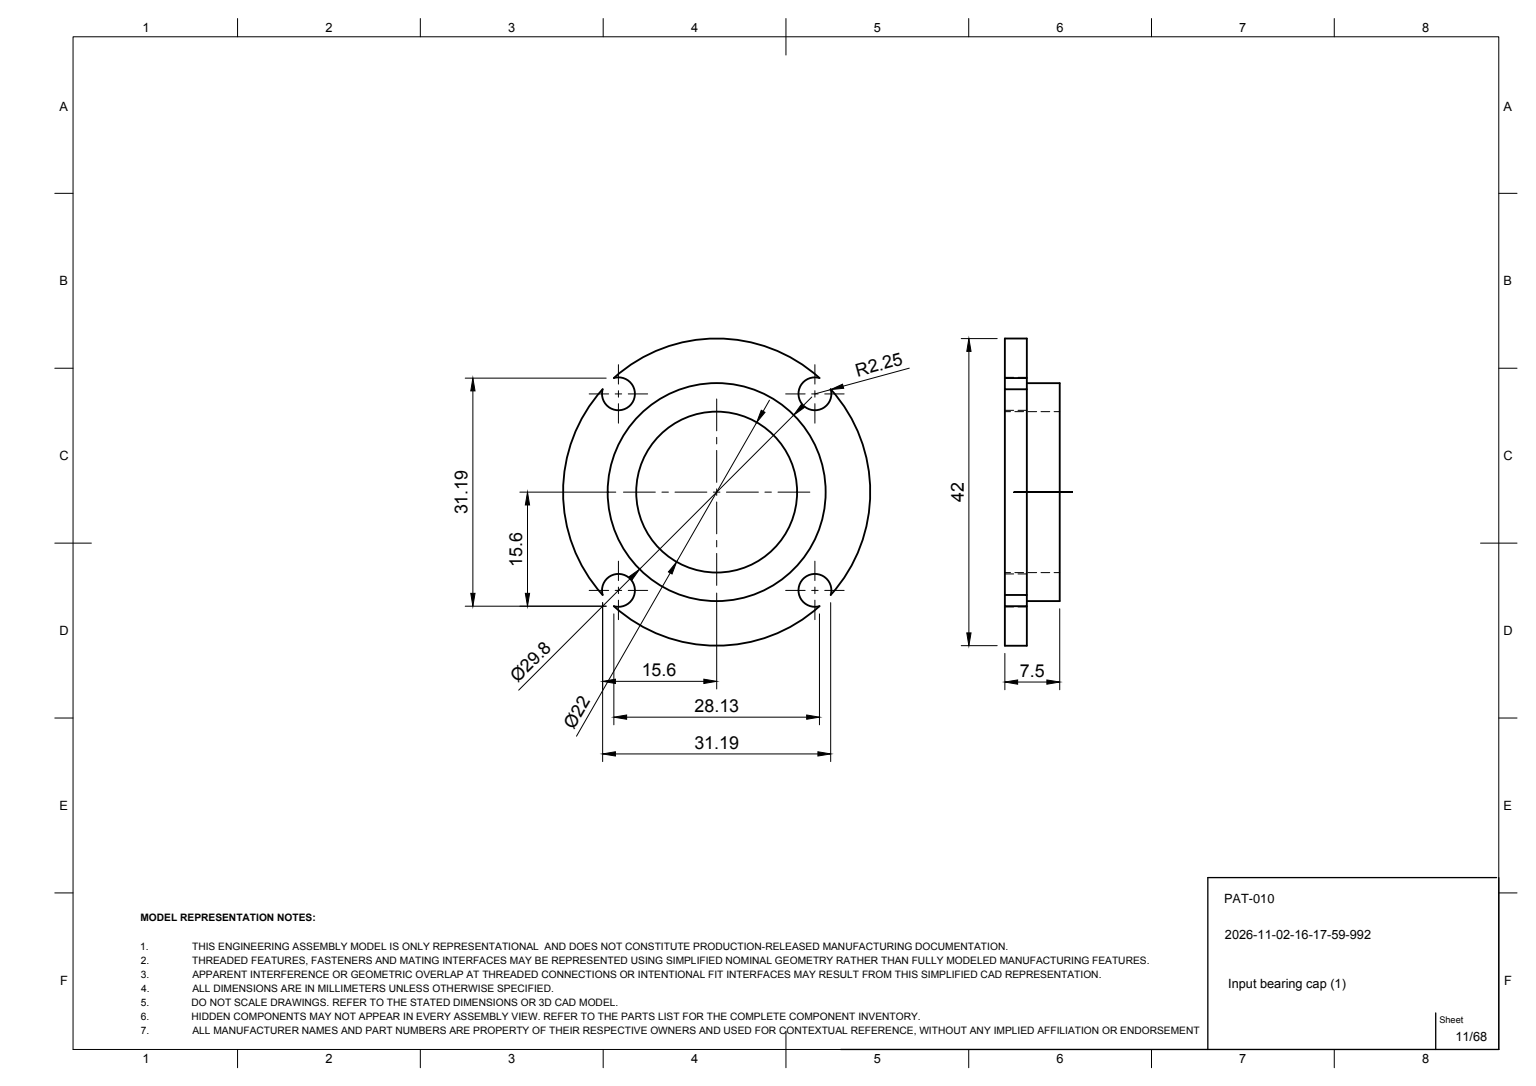
ISO-10303-21;
HEADER;
/* Generated by software containing ST-Developer
 * from STEP Tools, Inc. (www.steptools.com) 
 */

FILE_DESCRIPTION(
/* description */ ('Belt conveyor head drive unit'),
/* implementation_level */ '2;1');

FILE_NAME(
/* name */ 'Input bearing cap (1).step',
/* time_stamp */ '2026-10-28T03:26:19-07:00',
/* author */ (''),
/* organization */ (''),
/* preprocessor_version */ 'ST-DEVELOPER v20.2',
/* originating_system */ 'Autodesk Translation Framework v15.17.0.0',
/* authorisation */ '');

FILE_SCHEMA (('AUTOMOTIVE_DESIGN { 1 0 10303 214 3 1 1 }'));
ENDSEC;

DATA;
#10=MECHANICAL_DESIGN_GEOMETRIC_PRESENTATION_REPRESENTATION('',(#853),#27069);
#715=SHAPE_REPRESENTATION_RELATIONSHIP('SRR','None',#27359,#784);
#784=ADVANCED_BREP_SHAPE_REPRESENTATION('',(#938),#27001);
#853=STYLED_ITEM('',(#27797),#938);
#938=MANIFOLD_SOLID_BREP('Body1',#13718);
#1055=FACE_BOUND('',#2579,.T.);
#1056=FACE_BOUND('',#2586,.T.);
#1057=FACE_BOUND('',#2589,.T.);
#1332=PLANE('',#14771);
#1333=PLANE('',#14787);
#1334=PLANE('',#14791);
#1731=FACE_OUTER_BOUND('',#2574,.T.);
#1732=FACE_OUTER_BOUND('',#2575,.T.);
#1733=FACE_OUTER_BOUND('',#2576,.T.);
#1734=FACE_OUTER_BOUND('',#2577,.T.);
#1735=FACE_OUTER_BOUND('',#2578,.T.);
#1736=FACE_OUTER_BOUND('',#2580,.T.);
#1737=FACE_OUTER_BOUND('',#2581,.T.);
#1738=FACE_OUTER_BOUND('',#2582,.T.);
#1739=FACE_OUTER_BOUND('',#2583,.T.);
#1740=FACE_OUTER_BOUND('',#2584,.T.);
#1741=FACE_OUTER_BOUND('',#2585,.T.);
#1742=FACE_OUTER_BOUND('',#2587,.T.);
#1743=FACE_OUTER_BOUND('',#2588,.T.);
#2574=EDGE_LOOP('',(#9396,#9397,#9398,#9399));
#2575=EDGE_LOOP('',(#9400,#9401,#9402,#9403));
#2576=EDGE_LOOP('',(#9404,#9405,#9406,#9407));
#2577=EDGE_LOOP('',(#9408,#9409,#9410,#9411));
#2578=EDGE_LOOP('',(#9412,#9413,#9414,#9415,#9416,#9417,#9418,#9419));
#2579=EDGE_LOOP('',(#9420));
#2580=EDGE_LOOP('',(#9421,#9422,#9423,#9424));
#2581=EDGE_LOOP('',(#9425,#9426,#9427,#9428));
#2582=EDGE_LOOP('',(#9429,#9430,#9431,#9432));
#2583=EDGE_LOOP('',(#9433,#9434,#9435,#9436));
#2584=EDGE_LOOP('',(#9437,#9438,#9439,#9440));
#2585=EDGE_LOOP('',(#9441));
#2586=EDGE_LOOP('',(#9442));
#2587=EDGE_LOOP('',(#9443,#9444,#9445,#9446));
#2588=EDGE_LOOP('',(#9447,#9448,#9449,#9450,#9451,#9452,#9453,#9454));
#2589=EDGE_LOOP('',(#9455));
#3627=LINE('',#21445,#4419);
#3628=LINE('',#21449,#4420);
#3629=LINE('',#21454,#4421);
#3630=LINE('',#21458,#4422);
#3631=LINE('',#21463,#4423);
#3632=LINE('',#21467,#4424);
#3633=LINE('',#21472,#4425);
#3634=LINE('',#21476,#4426);
#3635=LINE('',#21495,#4427);
#3636=LINE('',#21503,#4428);
#4419=VECTOR('',#16959,1.);
#4420=VECTOR('',#16962,1.);
#4421=VECTOR('',#16967,1.);
#4422=VECTOR('',#16970,1.);
#4423=VECTOR('',#16975,1.);
#4424=VECTOR('',#16978,1.);
#4425=VECTOR('',#16983,1.);
#4426=VECTOR('',#16986,1.);
#4427=VECTOR('',#17019,1.49);
#4428=VECTOR('',#17030,1.1);
#5172=CIRCLE('',#14760,0.225);
#5173=CIRCLE('',#14761,0.225);
#5174=CIRCLE('',#14763,0.225);
#5175=CIRCLE('',#14764,0.225);
#5176=CIRCLE('',#14766,0.225);
#5177=CIRCLE('',#14767,0.225);
#5178=CIRCLE('',#14769,0.225);
#5179=CIRCLE('',#14770,0.225);
#5180=CIRCLE('',#14772,2.1);
#5181=CIRCLE('',#14773,2.1);
#5182=CIRCLE('',#14774,2.1);
#5183=CIRCLE('',#14775,2.1);
#5184=CIRCLE('',#14776,1.49);
#5185=CIRCLE('',#14778,2.1);
#5186=CIRCLE('',#14780,2.1);
#5187=CIRCLE('',#14782,2.1);
#5188=CIRCLE('',#14784,2.1);
#5189=CIRCLE('',#14786,1.49);
#5190=CIRCLE('',#14788,1.1);
#5191=CIRCLE('',#14790,1.1);
#6099=VERTEX_POINT('',#21443);
#6100=VERTEX_POINT('',#21444);
#6101=VERTEX_POINT('',#21446);
#6102=VERTEX_POINT('',#21448);
#6103=VERTEX_POINT('',#21452);
#6104=VERTEX_POINT('',#21453);
#6105=VERTEX_POINT('',#21455);
#6106=VERTEX_POINT('',#21457);
#6107=VERTEX_POINT('',#21461);
#6108=VERTEX_POINT('',#21462);
#6109=VERTEX_POINT('',#21464);
#6110=VERTEX_POINT('',#21466);
#6111=VERTEX_POINT('',#21470);
#6112=VERTEX_POINT('',#21471);
#6113=VERTEX_POINT('',#21473);
#6114=VERTEX_POINT('',#21475);
#6115=VERTEX_POINT('',#21483);
#6116=VERTEX_POINT('',#21494);
#6117=VERTEX_POINT('',#21498);
#6118=VERTEX_POINT('',#21501);
#7390=EDGE_CURVE('',#6099,#6100,#3627,.T.);
#7391=EDGE_CURVE('',#6101,#6099,#5172,.T.);
#7392=EDGE_CURVE('',#6102,#6101,#3628,.T.);
#7393=EDGE_CURVE('',#6100,#6102,#5173,.T.);
#7394=EDGE_CURVE('',#6103,#6104,#3629,.T.);
#7395=EDGE_CURVE('',#6105,#6103,#5174,.T.);
#7396=EDGE_CURVE('',#6106,#6105,#3630,.T.);
#7397=EDGE_CURVE('',#6104,#6106,#5175,.T.);
#7398=EDGE_CURVE('',#6107,#6108,#3631,.T.);
#7399=EDGE_CURVE('',#6109,#6107,#5176,.T.);
#7400=EDGE_CURVE('',#6110,#6109,#3632,.T.);
#7401=EDGE_CURVE('',#6108,#6110,#5177,.T.);
#7402=EDGE_CURVE('',#6111,#6112,#3633,.T.);
#7403=EDGE_CURVE('',#6113,#6111,#5178,.T.);
#7404=EDGE_CURVE('',#6114,#6113,#3634,.T.);
#7405=EDGE_CURVE('',#6112,#6114,#5179,.T.);
#7406=EDGE_CURVE('',#6113,#6099,#5180,.T.);
#7407=EDGE_CURVE('',#6109,#6111,#5181,.T.);
#7408=EDGE_CURVE('',#6105,#6107,#5182,.T.);
#7409=EDGE_CURVE('',#6101,#6103,#5183,.T.);
#7410=EDGE_CURVE('',#6115,#6115,#5184,.T.);
#7411=EDGE_CURVE('',#6110,#6112,#5185,.T.);
#7412=EDGE_CURVE('',#6106,#6108,#5186,.T.);
#7413=EDGE_CURVE('',#6114,#6100,#5187,.T.);
#7414=EDGE_CURVE('',#6102,#6104,#5188,.T.);
#7415=EDGE_CURVE('',#6115,#6116,#3635,.T.);
#7416=EDGE_CURVE('',#6116,#6116,#5189,.T.);
#7417=EDGE_CURVE('',#6117,#6117,#5190,.T.);
#7418=EDGE_CURVE('',#6118,#6118,#5191,.T.);
#7419=EDGE_CURVE('',#6118,#6117,#3636,.T.);
#9396=ORIENTED_EDGE('',*,*,#7390,.F.);
#9397=ORIENTED_EDGE('',*,*,#7391,.F.);
#9398=ORIENTED_EDGE('',*,*,#7392,.F.);
#9399=ORIENTED_EDGE('',*,*,#7393,.F.);
#9400=ORIENTED_EDGE('',*,*,#7394,.F.);
#9401=ORIENTED_EDGE('',*,*,#7395,.F.);
#9402=ORIENTED_EDGE('',*,*,#7396,.F.);
#9403=ORIENTED_EDGE('',*,*,#7397,.F.);
#9404=ORIENTED_EDGE('',*,*,#7398,.F.);
#9405=ORIENTED_EDGE('',*,*,#7399,.F.);
#9406=ORIENTED_EDGE('',*,*,#7400,.F.);
#9407=ORIENTED_EDGE('',*,*,#7401,.F.);
#9408=ORIENTED_EDGE('',*,*,#7402,.F.);
#9409=ORIENTED_EDGE('',*,*,#7403,.F.);
#9410=ORIENTED_EDGE('',*,*,#7404,.F.);
#9411=ORIENTED_EDGE('',*,*,#7405,.F.);
#9412=ORIENTED_EDGE('',*,*,#7391,.T.);
#9413=ORIENTED_EDGE('',*,*,#7406,.F.);
#9414=ORIENTED_EDGE('',*,*,#7403,.T.);
#9415=ORIENTED_EDGE('',*,*,#7407,.F.);
#9416=ORIENTED_EDGE('',*,*,#7399,.T.);
#9417=ORIENTED_EDGE('',*,*,#7408,.F.);
#9418=ORIENTED_EDGE('',*,*,#7395,.T.);
#9419=ORIENTED_EDGE('',*,*,#7409,.F.);
#9420=ORIENTED_EDGE('',*,*,#7410,.T.);
#9421=ORIENTED_EDGE('',*,*,#7400,.T.);
#9422=ORIENTED_EDGE('',*,*,#7407,.T.);
#9423=ORIENTED_EDGE('',*,*,#7402,.T.);
#9424=ORIENTED_EDGE('',*,*,#7411,.F.);
#9425=ORIENTED_EDGE('',*,*,#7396,.T.);
#9426=ORIENTED_EDGE('',*,*,#7408,.T.);
#9427=ORIENTED_EDGE('',*,*,#7398,.T.);
#9428=ORIENTED_EDGE('',*,*,#7412,.F.);
#9429=ORIENTED_EDGE('',*,*,#7390,.T.);
#9430=ORIENTED_EDGE('',*,*,#7413,.F.);
#9431=ORIENTED_EDGE('',*,*,#7404,.T.);
#9432=ORIENTED_EDGE('',*,*,#7406,.T.);
#9433=ORIENTED_EDGE('',*,*,#7392,.T.);
#9434=ORIENTED_EDGE('',*,*,#7409,.T.);
#9435=ORIENTED_EDGE('',*,*,#7394,.T.);
#9436=ORIENTED_EDGE('',*,*,#7414,.F.);
#9437=ORIENTED_EDGE('',*,*,#7410,.F.);
#9438=ORIENTED_EDGE('',*,*,#7415,.T.);
#9439=ORIENTED_EDGE('',*,*,#7416,.T.);
#9440=ORIENTED_EDGE('',*,*,#7415,.F.);
#9441=ORIENTED_EDGE('',*,*,#7416,.F.);
#9442=ORIENTED_EDGE('',*,*,#7417,.F.);
#9443=ORIENTED_EDGE('',*,*,#7418,.F.);
#9444=ORIENTED_EDGE('',*,*,#7419,.T.);
#9445=ORIENTED_EDGE('',*,*,#7417,.T.);
#9446=ORIENTED_EDGE('',*,*,#7419,.F.);
#9447=ORIENTED_EDGE('',*,*,#7393,.T.);
#9448=ORIENTED_EDGE('',*,*,#7414,.T.);
#9449=ORIENTED_EDGE('',*,*,#7397,.T.);
#9450=ORIENTED_EDGE('',*,*,#7412,.T.);
#9451=ORIENTED_EDGE('',*,*,#7401,.T.);
#9452=ORIENTED_EDGE('',*,*,#7411,.T.);
#9453=ORIENTED_EDGE('',*,*,#7405,.T.);
#9454=ORIENTED_EDGE('',*,*,#7413,.T.);
#9455=ORIENTED_EDGE('',*,*,#7418,.T.);
#12575=CYLINDRICAL_SURFACE('',#14759,0.225);
#12576=CYLINDRICAL_SURFACE('',#14762,0.225);
#12577=CYLINDRICAL_SURFACE('',#14765,0.225);
#12578=CYLINDRICAL_SURFACE('',#14768,0.225);
#12579=CYLINDRICAL_SURFACE('',#14777,2.1);
#12580=CYLINDRICAL_SURFACE('',#14779,2.1);
#12581=CYLINDRICAL_SURFACE('',#14781,2.1);
#12582=CYLINDRICAL_SURFACE('',#14783,2.1);
#12583=CYLINDRICAL_SURFACE('',#14785,1.49);
#12584=CYLINDRICAL_SURFACE('',#14789,1.1);
#13010=ADVANCED_FACE('',(#1731),#12575,.F.);
#13011=ADVANCED_FACE('',(#1732),#12576,.F.);
#13012=ADVANCED_FACE('',(#1733),#12577,.F.);
#13013=ADVANCED_FACE('',(#1734),#12578,.F.);
#13014=ADVANCED_FACE('',(#1735,#1055),#1332,.F.);
#13015=ADVANCED_FACE('',(#1736),#12579,.T.);
#13016=ADVANCED_FACE('',(#1737),#12580,.T.);
#13017=ADVANCED_FACE('',(#1738),#12581,.T.);
#13018=ADVANCED_FACE('',(#1739),#12582,.T.);
#13019=ADVANCED_FACE('',(#1740),#12583,.T.);
#13020=ADVANCED_FACE('',(#1741,#1056),#1333,.F.);
#13021=ADVANCED_FACE('',(#1742),#12584,.F.);
#13022=ADVANCED_FACE('',(#1743,#1057),#1334,.T.);
#13718=CLOSED_SHELL('',(#13010,#13011,#13012,#13013,#13014,#13015,#13016,
#13017,#13018,#13019,#13020,#13021,#13022));
#14758=AXIS2_PLACEMENT_3D('',#21441,#16955,#16956);
#14759=AXIS2_PLACEMENT_3D('',#21442,#16957,#16958);
#14760=AXIS2_PLACEMENT_3D('',#21447,#16960,#16961);
#14761=AXIS2_PLACEMENT_3D('',#21450,#16963,#16964);
#14762=AXIS2_PLACEMENT_3D('',#21451,#16965,#16966);
#14763=AXIS2_PLACEMENT_3D('',#21456,#16968,#16969);
#14764=AXIS2_PLACEMENT_3D('',#21459,#16971,#16972);
#14765=AXIS2_PLACEMENT_3D('',#21460,#16973,#16974);
#14766=AXIS2_PLACEMENT_3D('',#21465,#16976,#16977);
#14767=AXIS2_PLACEMENT_3D('',#21468,#16979,#16980);
#14768=AXIS2_PLACEMENT_3D('',#21469,#16981,#16982);
#14769=AXIS2_PLACEMENT_3D('',#21474,#16984,#16985);
#14770=AXIS2_PLACEMENT_3D('',#21477,#16987,#16988);
#14771=AXIS2_PLACEMENT_3D('',#21478,#16989,#16990);
#14772=AXIS2_PLACEMENT_3D('',#21479,#16991,#16992);
#14773=AXIS2_PLACEMENT_3D('',#21480,#16993,#16994);
#14774=AXIS2_PLACEMENT_3D('',#21481,#16995,#16996);
#14775=AXIS2_PLACEMENT_3D('',#21482,#16997,#16998);
#14776=AXIS2_PLACEMENT_3D('',#21484,#16999,#17000);
#14777=AXIS2_PLACEMENT_3D('',#21485,#17001,#17002);
#14778=AXIS2_PLACEMENT_3D('',#21486,#17003,#17004);
#14779=AXIS2_PLACEMENT_3D('',#21487,#17005,#17006);
#14780=AXIS2_PLACEMENT_3D('',#21488,#17007,#17008);
#14781=AXIS2_PLACEMENT_3D('',#21489,#17009,#17010);
#14782=AXIS2_PLACEMENT_3D('',#21490,#17011,#17012);
#14783=AXIS2_PLACEMENT_3D('',#21491,#17013,#17014);
#14784=AXIS2_PLACEMENT_3D('',#21492,#17015,#17016);
#14785=AXIS2_PLACEMENT_3D('',#21493,#17017,#17018);
#14786=AXIS2_PLACEMENT_3D('',#21496,#17020,#17021);
#14787=AXIS2_PLACEMENT_3D('',#21497,#17022,#17023);
#14788=AXIS2_PLACEMENT_3D('',#21499,#17024,#17025);
#14789=AXIS2_PLACEMENT_3D('',#21500,#17026,#17027);
#14790=AXIS2_PLACEMENT_3D('',#21502,#17028,#17029);
#14791=AXIS2_PLACEMENT_3D('',#21504,#17031,#17032);
#16955=DIRECTION('axis',(0.,0.,1.));
#16956=DIRECTION('refdir',(1.,0.,0.));
#16957=DIRECTION('center_axis',(0.,1.,0.));
#16958=DIRECTION('ref_axis',(0.707106781186546,0.,0.707106781186549));
#16959=DIRECTION('',(0.,1.,0.));
#16960=DIRECTION('center_axis',(0.,1.,0.));
#16961=DIRECTION('ref_axis',(1.,0.,0.));
#16962=DIRECTION('',(0.,-1.,0.));
#16963=DIRECTION('center_axis',(0.,-1.,0.));
#16964=DIRECTION('ref_axis',(1.,0.,0.));
#16965=DIRECTION('center_axis',(0.,1.,0.));
#16966=DIRECTION('ref_axis',(0.707106781186547,0.,-0.707106781186548));
#16967=DIRECTION('',(0.,1.,0.));
#16968=DIRECTION('center_axis',(0.,1.,0.));
#16969=DIRECTION('ref_axis',(1.,0.,0.));
#16970=DIRECTION('',(0.,-1.,0.));
#16971=DIRECTION('center_axis',(0.,-1.,0.));
#16972=DIRECTION('ref_axis',(1.,0.,0.));
#16973=DIRECTION('center_axis',(0.,1.,0.));
#16974=DIRECTION('ref_axis',(-0.707106781186552,0.,-0.707106781186543));
#16975=DIRECTION('',(0.,1.,0.));
#16976=DIRECTION('center_axis',(0.,1.,0.));
#16977=DIRECTION('ref_axis',(1.,0.,0.));
#16978=DIRECTION('',(0.,-1.,0.));
#16979=DIRECTION('center_axis',(0.,-1.,0.));
#16980=DIRECTION('ref_axis',(1.,0.,0.));
#16981=DIRECTION('center_axis',(0.,1.,0.));
#16982=DIRECTION('ref_axis',(-0.707106781186546,0.,0.707106781186549));
#16983=DIRECTION('',(0.,1.,0.));
#16984=DIRECTION('center_axis',(0.,1.,0.));
#16985=DIRECTION('ref_axis',(1.,0.,0.));
#16986=DIRECTION('',(0.,-1.,0.));
#16987=DIRECTION('center_axis',(0.,-1.,0.));
#16988=DIRECTION('ref_axis',(1.,0.,0.));
#16989=DIRECTION('center_axis',(0.,1.,0.));
#16990=DIRECTION('ref_axis',(1.,0.,0.));
#16991=DIRECTION('center_axis',(0.,1.,0.));
#16992=DIRECTION('ref_axis',(1.,0.,0.));
#16993=DIRECTION('center_axis',(0.,1.,0.));
#16994=DIRECTION('ref_axis',(1.,0.,0.));
#16995=DIRECTION('center_axis',(0.,1.,0.));
#16996=DIRECTION('ref_axis',(1.,0.,0.));
#16997=DIRECTION('center_axis',(0.,1.,0.));
#16998=DIRECTION('ref_axis',(1.,0.,0.));
#16999=DIRECTION('center_axis',(0.,1.,0.));
#17000=DIRECTION('ref_axis',(1.,0.,0.));
#17001=DIRECTION('center_axis',(0.,1.,0.));
#17002=DIRECTION('ref_axis',(1.,0.,0.));
#17003=DIRECTION('center_axis',(0.,1.,0.));
#17004=DIRECTION('ref_axis',(1.,0.,0.));
#17005=DIRECTION('center_axis',(0.,1.,0.));
#17006=DIRECTION('ref_axis',(1.,0.,0.));
#17007=DIRECTION('center_axis',(0.,1.,0.));
#17008=DIRECTION('ref_axis',(1.,0.,0.));
#17009=DIRECTION('center_axis',(0.,1.,0.));
#17010=DIRECTION('ref_axis',(1.,0.,0.));
#17011=DIRECTION('center_axis',(0.,1.,0.));
#17012=DIRECTION('ref_axis',(1.,0.,0.));
#17013=DIRECTION('center_axis',(0.,1.,0.));
#17014=DIRECTION('ref_axis',(-1.,0.,-1.22464679914735E-16));
#17015=DIRECTION('center_axis',(0.,1.,0.));
#17016=DIRECTION('ref_axis',(1.,0.,0.));
#17017=DIRECTION('center_axis',(0.,1.,0.));
#17018=DIRECTION('ref_axis',(1.,0.,0.));
#17019=DIRECTION('',(0.,-1.,0.));
#17020=DIRECTION('center_axis',(0.,1.,0.));
#17021=DIRECTION('ref_axis',(1.,0.,0.));
#17022=DIRECTION('center_axis',(0.,1.,0.));
#17023=DIRECTION('ref_axis',(1.,0.,0.));
#17024=DIRECTION('center_axis',(0.,-1.,0.));
#17025=DIRECTION('ref_axis',(1.,0.,0.));
#17026=DIRECTION('center_axis',(0.,1.,0.));
#17027=DIRECTION('ref_axis',(1.,0.,0.));
#17028=DIRECTION('center_axis',(0.,-1.,0.));
#17029=DIRECTION('ref_axis',(1.,0.,0.));
#17030=DIRECTION('',(0.,-1.,0.));
#17031=DIRECTION('center_axis',(0.,1.,0.));
#17032=DIRECTION('ref_axis',(1.,0.,0.));
#21441=CARTESIAN_POINT('',(0.,0.,0.));
#21442=CARTESIAN_POINT('Origin',(-1.34350288425444,1.7,5.65649711574556));
#21443=CARTESIAN_POINT('',(-1.40634555589641,1.8,5.4404512904656));
#21444=CARTESIAN_POINT('',(-1.40634555589641,2.1,5.4404512904656));
#21445=CARTESIAN_POINT('',(-1.40634555589641,1.7,5.4404512904656));
#21446=CARTESIAN_POINT('',(-1.5595487095344,1.8,5.59365444410359));
#21447=CARTESIAN_POINT('Origin',(-1.34350288425444,1.8,5.65649711574556));
#21448=CARTESIAN_POINT('',(-1.5595487095344,2.1,5.59365444410359));
#21449=CARTESIAN_POINT('',(-1.5595487095344,1.7,5.59365444410359));
#21450=CARTESIAN_POINT('Origin',(-1.34350288425444,2.1,5.65649711574556));
#21451=CARTESIAN_POINT('Origin',(-1.34350288425444,1.7,8.34350288425444));
#21452=CARTESIAN_POINT('',(-1.5595487095344,1.8,8.40634555589641));
#21453=CARTESIAN_POINT('',(-1.5595487095344,2.1,8.40634555589641));
#21454=CARTESIAN_POINT('',(-1.5595487095344,1.7,8.40634555589641));
#21455=CARTESIAN_POINT('',(-1.40634555589641,1.8,8.5595487095344));
#21456=CARTESIAN_POINT('Origin',(-1.34350288425444,1.8,8.34350288425444));
#21457=CARTESIAN_POINT('',(-1.40634555589641,2.1,8.5595487095344));
#21458=CARTESIAN_POINT('',(-1.40634555589641,1.7,8.5595487095344));
#21459=CARTESIAN_POINT('Origin',(-1.34350288425444,2.1,8.34350288425444));
#21460=CARTESIAN_POINT('Origin',(1.34350288425444,1.7,8.34350288425444));
#21461=CARTESIAN_POINT('',(1.40634555589641,1.8,8.5595487095344));
#21462=CARTESIAN_POINT('',(1.40634555589641,2.1,8.5595487095344));
#21463=CARTESIAN_POINT('',(1.40634555589641,1.7,8.5595487095344));
#21464=CARTESIAN_POINT('',(1.5595487095344,1.8,8.40634555589641));
#21465=CARTESIAN_POINT('Origin',(1.34350288425444,1.8,8.34350288425444));
#21466=CARTESIAN_POINT('',(1.5595487095344,2.1,8.40634555589641));
#21467=CARTESIAN_POINT('',(1.5595487095344,1.7,8.40634555589641));
#21468=CARTESIAN_POINT('Origin',(1.34350288425444,2.1,8.34350288425444));
#21469=CARTESIAN_POINT('Origin',(1.34350288425444,1.7,5.65649711574556));
#21470=CARTESIAN_POINT('',(1.5595487095344,1.8,5.59365444410359));
#21471=CARTESIAN_POINT('',(1.5595487095344,2.1,5.59365444410359));
#21472=CARTESIAN_POINT('',(1.5595487095344,1.7,5.59365444410359));
#21473=CARTESIAN_POINT('',(1.40634555589641,1.8,5.4404512904656));
#21474=CARTESIAN_POINT('Origin',(1.34350288425444,1.8,5.65649711574556));
#21475=CARTESIAN_POINT('',(1.40634555589641,2.1,5.4404512904656));
#21476=CARTESIAN_POINT('',(1.40634555589641,1.7,5.4404512904656));
#21477=CARTESIAN_POINT('Origin',(1.34350288425444,2.1,5.65649711574556));
#21478=CARTESIAN_POINT('Origin',(0.,1.8,7.));
#21479=CARTESIAN_POINT('Origin',(0.,1.8,7.));
#21480=CARTESIAN_POINT('Origin',(0.,1.8,7.));
#21481=CARTESIAN_POINT('Origin',(0.,1.8,7.));
#21482=CARTESIAN_POINT('Origin',(0.,1.8,7.));
#21483=CARTESIAN_POINT('',(-1.49,1.8,7.));
#21484=CARTESIAN_POINT('Origin',(0.,1.8,7.));
#21485=CARTESIAN_POINT('Origin',(0.,1.8,7.));
#21486=CARTESIAN_POINT('Origin',(0.,2.1,7.));
#21487=CARTESIAN_POINT('Origin',(0.,1.8,7.));
#21488=CARTESIAN_POINT('Origin',(0.,2.1,7.));
#21489=CARTESIAN_POINT('Origin',(0.,1.8,7.));
#21490=CARTESIAN_POINT('Origin',(0.,2.1,7.));
#21491=CARTESIAN_POINT('Origin',(0.,1.8,7.));
#21492=CARTESIAN_POINT('Origin',(0.,2.1,7.));
#21493=CARTESIAN_POINT('Origin',(0.,1.35,7.));
#21494=CARTESIAN_POINT('',(-1.49,1.35,7.));
#21495=CARTESIAN_POINT('',(-1.49,1.35,7.));
#21496=CARTESIAN_POINT('Origin',(0.,1.35,7.));
#21497=CARTESIAN_POINT('Origin',(0.,1.35,7.));
#21498=CARTESIAN_POINT('',(-1.1,1.35,7.));
#21499=CARTESIAN_POINT('Origin',(0.,1.35,7.));
#21500=CARTESIAN_POINT('Origin',(0.,1.8,7.));
#21501=CARTESIAN_POINT('',(-1.1,2.1,7.));
#21502=CARTESIAN_POINT('Origin',(0.,2.1,7.));
#21503=CARTESIAN_POINT('',(-1.1,1.8,7.));
#21504=CARTESIAN_POINT('Origin',(0.,2.1,7.));
#26924=UNCERTAINTY_MEASURE_WITH_UNIT(LENGTH_MEASURE(0.001),#27070,
'DISTANCE_ACCURACY_VALUE',
'Maximum model space distance between geometric entities at asserted c
onnectivities');
#26992=UNCERTAINTY_MEASURE_WITH_UNIT(LENGTH_MEASURE(0.001),#27070,
'DISTANCE_ACCURACY_VALUE',
'Maximum model space distance between geometric entities at asserted c
onnectivities');
#27001=(
GEOMETRIC_REPRESENTATION_CONTEXT(3)
GLOBAL_UNCERTAINTY_ASSIGNED_CONTEXT((#26924))
GLOBAL_UNIT_ASSIGNED_CONTEXT((#27070,#27072,#27073))
REPRESENTATION_CONTEXT('','3D')
);
#27069=(
GEOMETRIC_REPRESENTATION_CONTEXT(3)
GLOBAL_UNCERTAINTY_ASSIGNED_CONTEXT((#26992))
GLOBAL_UNIT_ASSIGNED_CONTEXT((#27070,#27072,#27073))
REPRESENTATION_CONTEXT('','3D')
);
#27070=(
LENGTH_UNIT()
NAMED_UNIT(*)
SI_UNIT(.CENTI.,.METRE.)
);
#27072=(
NAMED_UNIT(*)
PLANE_ANGLE_UNIT()
SI_UNIT($,.RADIAN.)
);
#27073=(
NAMED_UNIT(*)
SI_UNIT($,.STERADIAN.)
SOLID_ANGLE_UNIT()
);
#27082=SHAPE_DEFINITION_REPRESENTATION(#27158,#27359);
#27158=PRODUCT_DEFINITION_SHAPE('',$,#27436);
#27359=SHAPE_REPRESENTATION('',(#14758),#27001);
#27427=PRODUCT_DEFINITION_CONTEXT('part definition',#27657,'design');
#27436=PRODUCT_DEFINITION('Input bearing cap (1)','Input bearing cap (1)',
#27512,#27427);
#27512=PRODUCT_DEFINITION_FORMATION('',$,#27667);
#27657=APPLICATION_CONTEXT(
'Core Data for Automotive Mechanical Design Process');
#27658=PRODUCT_CONTEXT('part definition',#27657,'mechanical');
#27667=PRODUCT('Input bearing cap (1)','Input bearing cap (1)',
'Input bearing cap (1)',(#27658));
#27791=COLOUR_RGB('Grey',0.48,0.52,0.57);
#27792=FILL_AREA_STYLE_COLOUR('',#27791);
#27793=FILL_AREA_STYLE('',(#27792));
#27794=SURFACE_STYLE_FILL_AREA(#27793);
#27795=SURFACE_SIDE_STYLE('',(#27794));
#27796=SURFACE_STYLE_USAGE(.BOTH.,#27795);
#27797=PRESENTATION_STYLE_ASSIGNMENT((#27796));
ENDSEC;
END-ISO-10303-21;
